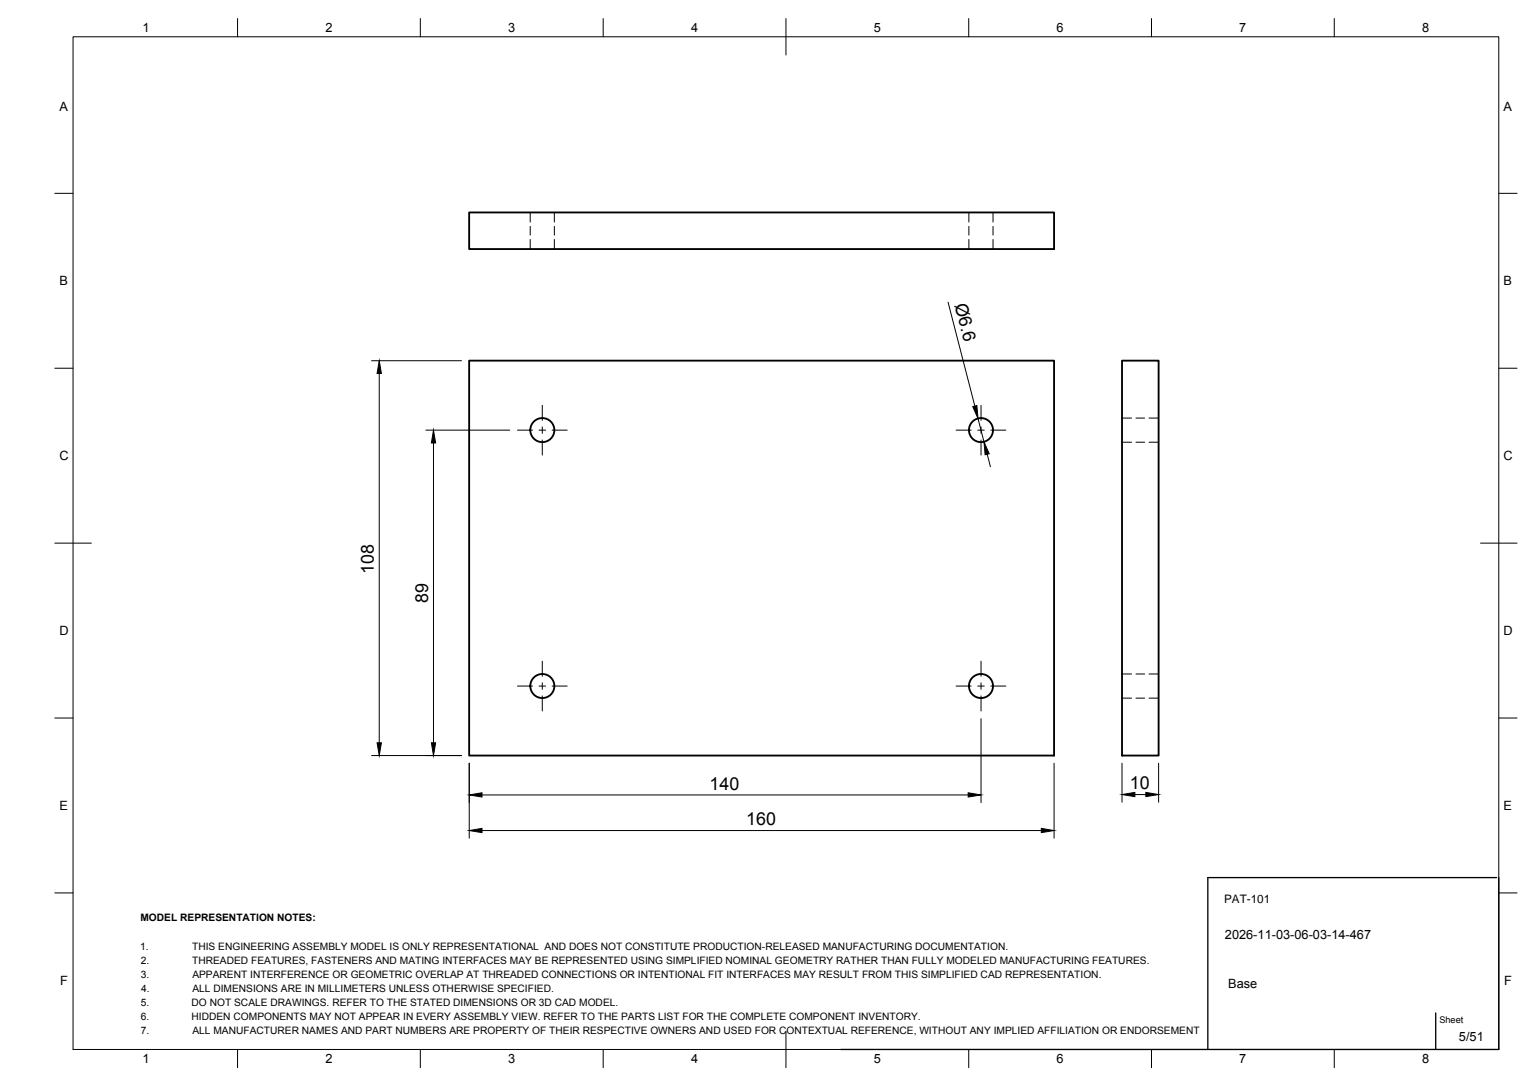
ISO-10303-21;
HEADER;
/* Generated by software containing ST-Developer
 * from STEP Tools, Inc. (www.steptools.com) 
 */

FILE_DESCRIPTION(
/* description */ ('Spur gear reduction stage 2-1 on bearing plates'),
/* implementation_level */ '2;1');

FILE_NAME(
/* name */ 'Base.step',
/* time_stamp */ '2026-10-28T03:22:07-07:00',
/* author */ (''),
/* organization */ (''),
/* preprocessor_version */ 'ST-DEVELOPER v20.2',
/* originating_system */ 'Autodesk Translation Framework v15.17.0.0',
/* authorisation */ '');

FILE_SCHEMA (('AUTOMOTIVE_DESIGN { 1 0 10303 214 3 1 1 }'));
ENDSEC;

DATA;
#10=MECHANICAL_DESIGN_GEOMETRIC_PRESENTATION_REPRESENTATION('',(#947),#53909);
#861=SHAPE_REPRESENTATION_RELATIONSHIP('SRR','None',#54088,#904);
#904=ADVANCED_BREP_SHAPE_REPRESENTATION('',(#1005),#53862);
#947=STYLED_ITEM('',(#54376),#1005);
#1005=MANIFOLD_SOLID_BREP('Body1',#11271);
#1060=FACE_BOUND('',#2160,.T.);
#1061=FACE_BOUND('',#2161,.T.);
#1062=FACE_BOUND('',#2162,.T.);
#1063=FACE_BOUND('',#2163,.T.);
#1064=FACE_BOUND('',#2165,.T.);
#1065=FACE_BOUND('',#2166,.T.);
#1066=FACE_BOUND('',#2167,.T.);
#1067=FACE_BOUND('',#2168,.T.);
#1238=PLANE('',#11821);
#1239=PLANE('',#11822);
#1240=PLANE('',#11823);
#1241=PLANE('',#11824);
#1242=PLANE('',#11825);
#1243=PLANE('',#11826);
#1503=FACE_OUTER_BOUND('',#2151,.T.);
#1504=FACE_OUTER_BOUND('',#2152,.T.);
#1505=FACE_OUTER_BOUND('',#2153,.T.);
#1506=FACE_OUTER_BOUND('',#2154,.T.);
#1507=FACE_OUTER_BOUND('',#2155,.T.);
#1508=FACE_OUTER_BOUND('',#2156,.T.);
#1509=FACE_OUTER_BOUND('',#2157,.T.);
#1510=FACE_OUTER_BOUND('',#2158,.T.);
#1511=FACE_OUTER_BOUND('',#2159,.T.);
#1512=FACE_OUTER_BOUND('',#2164,.T.);
#2151=EDGE_LOOP('',(#7352,#7353,#7354,#7355));
#2152=EDGE_LOOP('',(#7356,#7357,#7358,#7359));
#2153=EDGE_LOOP('',(#7360,#7361,#7362,#7363));
#2154=EDGE_LOOP('',(#7364,#7365,#7366,#7367));
#2155=EDGE_LOOP('',(#7368,#7369,#7370,#7371));
#2156=EDGE_LOOP('',(#7372,#7373,#7374,#7375));
#2157=EDGE_LOOP('',(#7376,#7377,#7378,#7379));
#2158=EDGE_LOOP('',(#7380,#7381,#7382,#7383));
#2159=EDGE_LOOP('',(#7384,#7385,#7386,#7387));
#2160=EDGE_LOOP('',(#7388));
#2161=EDGE_LOOP('',(#7389));
#2162=EDGE_LOOP('',(#7390));
#2163=EDGE_LOOP('',(#7391));
#2164=EDGE_LOOP('',(#7392,#7393,#7394,#7395));
#2165=EDGE_LOOP('',(#7396));
#2166=EDGE_LOOP('',(#7397));
#2167=EDGE_LOOP('',(#7398));
#2168=EDGE_LOOP('',(#7399));
#2977=LINE('',#15982,#3618);
#2978=LINE('',#15988,#3619);
#2979=LINE('',#15994,#3620);
#2980=LINE('',#16000,#3621);
#2981=LINE('',#16005,#3622);
#2982=LINE('',#16007,#3623);
#2983=LINE('',#16009,#3624);
#2984=LINE('',#16010,#3625);
#2985=LINE('',#16013,#3626);
#2986=LINE('',#16015,#3627);
#2987=LINE('',#16016,#3628);
#2988=LINE('',#16019,#3629);
#2989=LINE('',#16021,#3630);
#2990=LINE('',#16022,#3631);
#2991=LINE('',#16024,#3632);
#2992=LINE('',#16025,#3633);
#3618=VECTOR('',#12992,0.33);
#3619=VECTOR('',#12999,0.33);
#3620=VECTOR('',#13006,0.33);
#3621=VECTOR('',#13013,0.33);
#3622=VECTOR('',#13018,1.);
#3623=VECTOR('',#13019,1.);
#3624=VECTOR('',#13020,1.);
#3625=VECTOR('',#13021,1.);
#3626=VECTOR('',#13024,1.);
#3627=VECTOR('',#13025,1.);
#3628=VECTOR('',#13026,1.);
#3629=VECTOR('',#13029,1.);
#3630=VECTOR('',#13030,1.);
#3631=VECTOR('',#13031,1.);
#3632=VECTOR('',#13034,1.);
#3633=VECTOR('',#13035,1.);
#4259=CIRCLE('',#11810,0.33);
#4260=CIRCLE('',#11811,0.33);
#4261=CIRCLE('',#11813,0.33);
#4262=CIRCLE('',#11814,0.33);
#4263=CIRCLE('',#11816,0.33);
#4264=CIRCLE('',#11817,0.33);
#4265=CIRCLE('',#11819,0.33);
#4266=CIRCLE('',#11820,0.33);
#4784=VERTEX_POINT('',#15979);
#4785=VERTEX_POINT('',#15981);
#4786=VERTEX_POINT('',#15985);
#4787=VERTEX_POINT('',#15987);
#4788=VERTEX_POINT('',#15991);
#4789=VERTEX_POINT('',#15993);
#4790=VERTEX_POINT('',#15997);
#4791=VERTEX_POINT('',#15999);
#4792=VERTEX_POINT('',#16003);
#4793=VERTEX_POINT('',#16004);
#4794=VERTEX_POINT('',#16006);
#4795=VERTEX_POINT('',#16008);
#4796=VERTEX_POINT('',#16012);
#4797=VERTEX_POINT('',#16014);
#4798=VERTEX_POINT('',#16018);
#4799=VERTEX_POINT('',#16020);
#5818=EDGE_CURVE('',#4784,#4784,#4259,.T.);
#5819=EDGE_CURVE('',#4784,#4785,#2977,.T.);
#5820=EDGE_CURVE('',#4785,#4785,#4260,.T.);
#5821=EDGE_CURVE('',#4786,#4786,#4261,.T.);
#5822=EDGE_CURVE('',#4786,#4787,#2978,.T.);
#5823=EDGE_CURVE('',#4787,#4787,#4262,.T.);
#5824=EDGE_CURVE('',#4788,#4788,#4263,.T.);
#5825=EDGE_CURVE('',#4788,#4789,#2979,.T.);
#5826=EDGE_CURVE('',#4789,#4789,#4264,.T.);
#5827=EDGE_CURVE('',#4790,#4790,#4265,.T.);
#5828=EDGE_CURVE('',#4790,#4791,#2980,.T.);
#5829=EDGE_CURVE('',#4791,#4791,#4266,.T.);
#5830=EDGE_CURVE('',#4792,#4793,#2981,.T.);
#5831=EDGE_CURVE('',#4793,#4794,#2982,.T.);
#5832=EDGE_CURVE('',#4795,#4794,#2983,.T.);
#5833=EDGE_CURVE('',#4792,#4795,#2984,.T.);
#5834=EDGE_CURVE('',#4796,#4792,#2985,.T.);
#5835=EDGE_CURVE('',#4797,#4795,#2986,.T.);
#5836=EDGE_CURVE('',#4796,#4797,#2987,.T.);
#5837=EDGE_CURVE('',#4798,#4796,#2988,.T.);
#5838=EDGE_CURVE('',#4799,#4797,#2989,.T.);
#5839=EDGE_CURVE('',#4798,#4799,#2990,.T.);
#5840=EDGE_CURVE('',#4793,#4798,#2991,.T.);
#5841=EDGE_CURVE('',#4794,#4799,#2992,.T.);
#7352=ORIENTED_EDGE('',*,*,#5818,.F.);
#7353=ORIENTED_EDGE('',*,*,#5819,.T.);
#7354=ORIENTED_EDGE('',*,*,#5820,.F.);
#7355=ORIENTED_EDGE('',*,*,#5819,.F.);
#7356=ORIENTED_EDGE('',*,*,#5821,.F.);
#7357=ORIENTED_EDGE('',*,*,#5822,.T.);
#7358=ORIENTED_EDGE('',*,*,#5823,.F.);
#7359=ORIENTED_EDGE('',*,*,#5822,.F.);
#7360=ORIENTED_EDGE('',*,*,#5824,.F.);
#7361=ORIENTED_EDGE('',*,*,#5825,.T.);
#7362=ORIENTED_EDGE('',*,*,#5826,.F.);
#7363=ORIENTED_EDGE('',*,*,#5825,.F.);
#7364=ORIENTED_EDGE('',*,*,#5827,.F.);
#7365=ORIENTED_EDGE('',*,*,#5828,.T.);
#7366=ORIENTED_EDGE('',*,*,#5829,.F.);
#7367=ORIENTED_EDGE('',*,*,#5828,.F.);
#7368=ORIENTED_EDGE('',*,*,#5830,.T.);
#7369=ORIENTED_EDGE('',*,*,#5831,.T.);
#7370=ORIENTED_EDGE('',*,*,#5832,.F.);
#7371=ORIENTED_EDGE('',*,*,#5833,.F.);
#7372=ORIENTED_EDGE('',*,*,#5834,.T.);
#7373=ORIENTED_EDGE('',*,*,#5833,.T.);
#7374=ORIENTED_EDGE('',*,*,#5835,.F.);
#7375=ORIENTED_EDGE('',*,*,#5836,.F.);
#7376=ORIENTED_EDGE('',*,*,#5837,.T.);
#7377=ORIENTED_EDGE('',*,*,#5836,.T.);
#7378=ORIENTED_EDGE('',*,*,#5838,.F.);
#7379=ORIENTED_EDGE('',*,*,#5839,.F.);
#7380=ORIENTED_EDGE('',*,*,#5840,.T.);
#7381=ORIENTED_EDGE('',*,*,#5839,.T.);
#7382=ORIENTED_EDGE('',*,*,#5841,.F.);
#7383=ORIENTED_EDGE('',*,*,#5831,.F.);
#7384=ORIENTED_EDGE('',*,*,#5841,.T.);
#7385=ORIENTED_EDGE('',*,*,#5838,.T.);
#7386=ORIENTED_EDGE('',*,*,#5835,.T.);
#7387=ORIENTED_EDGE('',*,*,#5832,.T.);
#7388=ORIENTED_EDGE('',*,*,#5820,.T.);
#7389=ORIENTED_EDGE('',*,*,#5823,.T.);
#7390=ORIENTED_EDGE('',*,*,#5826,.T.);
#7391=ORIENTED_EDGE('',*,*,#5829,.T.);
#7392=ORIENTED_EDGE('',*,*,#5840,.F.);
#7393=ORIENTED_EDGE('',*,*,#5830,.F.);
#7394=ORIENTED_EDGE('',*,*,#5834,.F.);
#7395=ORIENTED_EDGE('',*,*,#5837,.F.);
#7396=ORIENTED_EDGE('',*,*,#5818,.T.);
#7397=ORIENTED_EDGE('',*,*,#5821,.T.);
#7398=ORIENTED_EDGE('',*,*,#5824,.T.);
#7399=ORIENTED_EDGE('',*,*,#5827,.T.);
#10420=CYLINDRICAL_SURFACE('',#11809,0.33);
#10421=CYLINDRICAL_SURFACE('',#11812,0.33);
#10422=CYLINDRICAL_SURFACE('',#11815,0.33);
#10423=CYLINDRICAL_SURFACE('',#11818,0.33);
#10623=ADVANCED_FACE('',(#1503),#10420,.F.);
#10624=ADVANCED_FACE('',(#1504),#10421,.F.);
#10625=ADVANCED_FACE('',(#1505),#10422,.F.);
#10626=ADVANCED_FACE('',(#1506),#10423,.F.);
#10627=ADVANCED_FACE('',(#1507),#1238,.T.);
#10628=ADVANCED_FACE('',(#1508),#1239,.T.);
#10629=ADVANCED_FACE('',(#1509),#1240,.T.);
#10630=ADVANCED_FACE('',(#1510),#1241,.T.);
#10631=ADVANCED_FACE('',(#1511,#1060,#1061,#1062,#1063),#1242,.T.);
#10632=ADVANCED_FACE('',(#1512,#1064,#1065,#1066,#1067),#1243,.F.);
#11271=CLOSED_SHELL('',(#10623,#10624,#10625,#10626,#10627,#10628,#10629,
#10630,#10631,#10632));
#11808=AXIS2_PLACEMENT_3D('',#15977,#12986,#12987);
#11809=AXIS2_PLACEMENT_3D('',#15978,#12988,#12989);
#11810=AXIS2_PLACEMENT_3D('',#15980,#12990,#12991);
#11811=AXIS2_PLACEMENT_3D('',#15983,#12993,#12994);
#11812=AXIS2_PLACEMENT_3D('',#15984,#12995,#12996);
#11813=AXIS2_PLACEMENT_3D('',#15986,#12997,#12998);
#11814=AXIS2_PLACEMENT_3D('',#15989,#13000,#13001);
#11815=AXIS2_PLACEMENT_3D('',#15990,#13002,#13003);
#11816=AXIS2_PLACEMENT_3D('',#15992,#13004,#13005);
#11817=AXIS2_PLACEMENT_3D('',#15995,#13007,#13008);
#11818=AXIS2_PLACEMENT_3D('',#15996,#13009,#13010);
#11819=AXIS2_PLACEMENT_3D('',#15998,#13011,#13012);
#11820=AXIS2_PLACEMENT_3D('',#16001,#13014,#13015);
#11821=AXIS2_PLACEMENT_3D('',#16002,#13016,#13017);
#11822=AXIS2_PLACEMENT_3D('',#16011,#13022,#13023);
#11823=AXIS2_PLACEMENT_3D('',#16017,#13027,#13028);
#11824=AXIS2_PLACEMENT_3D('',#16023,#13032,#13033);
#11825=AXIS2_PLACEMENT_3D('',#16026,#13036,#13037);
#11826=AXIS2_PLACEMENT_3D('',#16027,#13038,#13039);
#12986=DIRECTION('axis',(0.,0.,1.));
#12987=DIRECTION('refdir',(1.,0.,0.));
#12988=DIRECTION('center_axis',(0.,0.,1.));
#12989=DIRECTION('ref_axis',(1.,0.,0.));
#12990=DIRECTION('center_axis',(0.,0.,1.));
#12991=DIRECTION('ref_axis',(1.,0.,0.));
#12992=DIRECTION('',(0.,0.,1.));
#12993=DIRECTION('center_axis',(0.,0.,-1.));
#12994=DIRECTION('ref_axis',(1.,0.,0.));
#12995=DIRECTION('center_axis',(0.,0.,1.));
#12996=DIRECTION('ref_axis',(1.,0.,0.));
#12997=DIRECTION('center_axis',(0.,0.,1.));
#12998=DIRECTION('ref_axis',(1.,0.,0.));
#12999=DIRECTION('',(0.,0.,1.));
#13000=DIRECTION('center_axis',(0.,0.,-1.));
#13001=DIRECTION('ref_axis',(1.,0.,0.));
#13002=DIRECTION('center_axis',(0.,0.,1.));
#13003=DIRECTION('ref_axis',(1.,0.,0.));
#13004=DIRECTION('center_axis',(0.,0.,1.));
#13005=DIRECTION('ref_axis',(1.,0.,0.));
#13006=DIRECTION('',(0.,0.,1.));
#13007=DIRECTION('center_axis',(0.,0.,-1.));
#13008=DIRECTION('ref_axis',(1.,0.,0.));
#13009=DIRECTION('center_axis',(0.,0.,1.));
#13010=DIRECTION('ref_axis',(1.,0.,0.));
#13011=DIRECTION('center_axis',(0.,0.,1.));
#13012=DIRECTION('ref_axis',(1.,0.,0.));
#13013=DIRECTION('',(0.,0.,1.));
#13014=DIRECTION('center_axis',(0.,0.,-1.));
#13015=DIRECTION('ref_axis',(1.,0.,0.));
#13016=DIRECTION('center_axis',(0.,1.,0.));
#13017=DIRECTION('ref_axis',(-1.,0.,0.));
#13018=DIRECTION('',(-1.,0.,0.));
#13019=DIRECTION('',(0.,0.,1.));
#13020=DIRECTION('',(-1.,0.,0.));
#13021=DIRECTION('',(0.,0.,1.));
#13022=DIRECTION('center_axis',(1.,0.,0.));
#13023=DIRECTION('ref_axis',(0.,1.,0.));
#13024=DIRECTION('',(0.,1.,0.));
#13025=DIRECTION('',(0.,1.,0.));
#13026=DIRECTION('',(0.,0.,1.));
#13027=DIRECTION('center_axis',(0.,-1.,0.));
#13028=DIRECTION('ref_axis',(1.,0.,0.));
#13029=DIRECTION('',(1.,0.,0.));
#13030=DIRECTION('',(1.,0.,0.));
#13031=DIRECTION('',(0.,0.,1.));
#13032=DIRECTION('center_axis',(-1.,0.,0.));
#13033=DIRECTION('ref_axis',(0.,-1.,0.));
#13034=DIRECTION('',(0.,-1.,0.));
#13035=DIRECTION('',(0.,-1.,0.));
#13036=DIRECTION('center_axis',(0.,0.,1.));
#13037=DIRECTION('ref_axis',(1.,0.,0.));
#13038=DIRECTION('center_axis',(0.,0.,1.));
#13039=DIRECTION('ref_axis',(1.,0.,0.));
#15977=CARTESIAN_POINT('',(0.,0.,0.));
#15978=CARTESIAN_POINT('Origin',(10.,-3.5,-1.1));
#15979=CARTESIAN_POINT('',(9.67,-3.5,-1.));
#15980=CARTESIAN_POINT('Origin',(10.,-3.5,-1.));
#15981=CARTESIAN_POINT('',(9.67,-3.5,0.));
#15982=CARTESIAN_POINT('',(9.67,-3.5,-1.1));
#15983=CARTESIAN_POINT('Origin',(10.,-3.5,0.));
#15984=CARTESIAN_POINT('Origin',(-2.,3.5,-1.1));
#15985=CARTESIAN_POINT('',(-2.33,3.5,-1.));
#15986=CARTESIAN_POINT('Origin',(-2.,3.5,-1.));
#15987=CARTESIAN_POINT('',(-2.33,3.5,0.));
#15988=CARTESIAN_POINT('',(-2.33,3.5,-1.1));
#15989=CARTESIAN_POINT('Origin',(-2.,3.5,0.));
#15990=CARTESIAN_POINT('Origin',(-2.,-3.5,-1.1));
#15991=CARTESIAN_POINT('',(-2.33,-3.5,-1.));
#15992=CARTESIAN_POINT('Origin',(-2.,-3.5,-1.));
#15993=CARTESIAN_POINT('',(-2.33,-3.5,0.));
#15994=CARTESIAN_POINT('',(-2.33,-3.5,-1.1));
#15995=CARTESIAN_POINT('Origin',(-2.,-3.5,0.));
#15996=CARTESIAN_POINT('Origin',(10.,3.5,-1.1));
#15997=CARTESIAN_POINT('',(9.67,3.5,-1.));
#15998=CARTESIAN_POINT('Origin',(10.,3.5,-1.));
#15999=CARTESIAN_POINT('',(9.67,3.5,0.));
#16000=CARTESIAN_POINT('',(9.67,3.5,-1.1));
#16001=CARTESIAN_POINT('Origin',(10.,3.5,0.));
#16002=CARTESIAN_POINT('Origin',(12.,5.4,-1.));
#16003=CARTESIAN_POINT('',(12.,5.4,-1.));
#16004=CARTESIAN_POINT('',(-4.,5.4,-1.));
#16005=CARTESIAN_POINT('',(12.,5.4,-1.));
#16006=CARTESIAN_POINT('',(-4.,5.4,0.));
#16007=CARTESIAN_POINT('',(-4.,5.4,-1.));
#16008=CARTESIAN_POINT('',(12.,5.4,0.));
#16009=CARTESIAN_POINT('',(12.,5.4,0.));
#16010=CARTESIAN_POINT('',(12.,5.4,-1.));
#16011=CARTESIAN_POINT('Origin',(12.,-5.4,-1.));
#16012=CARTESIAN_POINT('',(12.,-5.4,-1.));
#16013=CARTESIAN_POINT('',(12.,-5.4,-1.));
#16014=CARTESIAN_POINT('',(12.,-5.4,0.));
#16015=CARTESIAN_POINT('',(12.,-5.4,0.));
#16016=CARTESIAN_POINT('',(12.,-5.4,-1.));
#16017=CARTESIAN_POINT('Origin',(-4.,-5.4,-1.));
#16018=CARTESIAN_POINT('',(-4.,-5.4,-1.));
#16019=CARTESIAN_POINT('',(-4.,-5.4,-1.));
#16020=CARTESIAN_POINT('',(-4.,-5.4,0.));
#16021=CARTESIAN_POINT('',(-4.,-5.4,0.));
#16022=CARTESIAN_POINT('',(-4.,-5.4,-1.));
#16023=CARTESIAN_POINT('Origin',(-4.,5.4,-1.));
#16024=CARTESIAN_POINT('',(-4.,5.4,-1.));
#16025=CARTESIAN_POINT('',(-4.,5.4,0.));
#16026=CARTESIAN_POINT('Origin',(4.,0.,0.));
#16027=CARTESIAN_POINT('Origin',(4.,0.,-1.));
#53812=UNCERTAINTY_MEASURE_WITH_UNIT(LENGTH_MEASURE(0.001),#53910,
'DISTANCE_ACCURACY_VALUE',
'Maximum model space distance between geometric entities at asserted c
onnectivities');
#53859=UNCERTAINTY_MEASURE_WITH_UNIT(LENGTH_MEASURE(0.001),#53910,
'DISTANCE_ACCURACY_VALUE',
'Maximum model space distance between geometric entities at asserted c
onnectivities');
#53862=(
GEOMETRIC_REPRESENTATION_CONTEXT(3)
GLOBAL_UNCERTAINTY_ASSIGNED_CONTEXT((#53812))
GLOBAL_UNIT_ASSIGNED_CONTEXT((#53910,#53912,#53913))
REPRESENTATION_CONTEXT('','3D')
);
#53909=(
GEOMETRIC_REPRESENTATION_CONTEXT(3)
GLOBAL_UNCERTAINTY_ASSIGNED_CONTEXT((#53859))
GLOBAL_UNIT_ASSIGNED_CONTEXT((#53910,#53912,#53913))
REPRESENTATION_CONTEXT('','3D')
);
#53910=(
LENGTH_UNIT()
NAMED_UNIT(*)
SI_UNIT(.CENTI.,.METRE.)
);
#53912=(
NAMED_UNIT(*)
PLANE_ANGLE_UNIT()
SI_UNIT($,.RADIAN.)
);
#53913=(
NAMED_UNIT(*)
SI_UNIT($,.STERADIAN.)
SOLID_ANGLE_UNIT()
);
#53916=SHAPE_DEFINITION_REPRESENTATION(#53965,#54088);
#53965=PRODUCT_DEFINITION_SHAPE('',$,#54138);
#54088=SHAPE_REPRESENTATION('',(#11808),#53862);
#54135=PRODUCT_DEFINITION_CONTEXT('part definition',#54284,'design');
#54138=PRODUCT_DEFINITION('Base','Base',#54187,#54135);
#54187=PRODUCT_DEFINITION_FORMATION('',$,#54288);
#54284=APPLICATION_CONTEXT(
'Core Data for Automotive Mechanical Design Process');
#54285=PRODUCT_CONTEXT('part definition',#54284,'mechanical');
#54288=PRODUCT('Base','Base','Base',(#54285));
#54370=COLOUR_RGB('Dark Blue',0.08,0.2,0.34);
#54371=FILL_AREA_STYLE_COLOUR('',#54370);
#54372=FILL_AREA_STYLE('',(#54371));
#54373=SURFACE_STYLE_FILL_AREA(#54372);
#54374=SURFACE_SIDE_STYLE('',(#54373));
#54375=SURFACE_STYLE_USAGE(.BOTH.,#54374);
#54376=PRESENTATION_STYLE_ASSIGNMENT((#54375));
ENDSEC;
END-ISO-10303-21;
